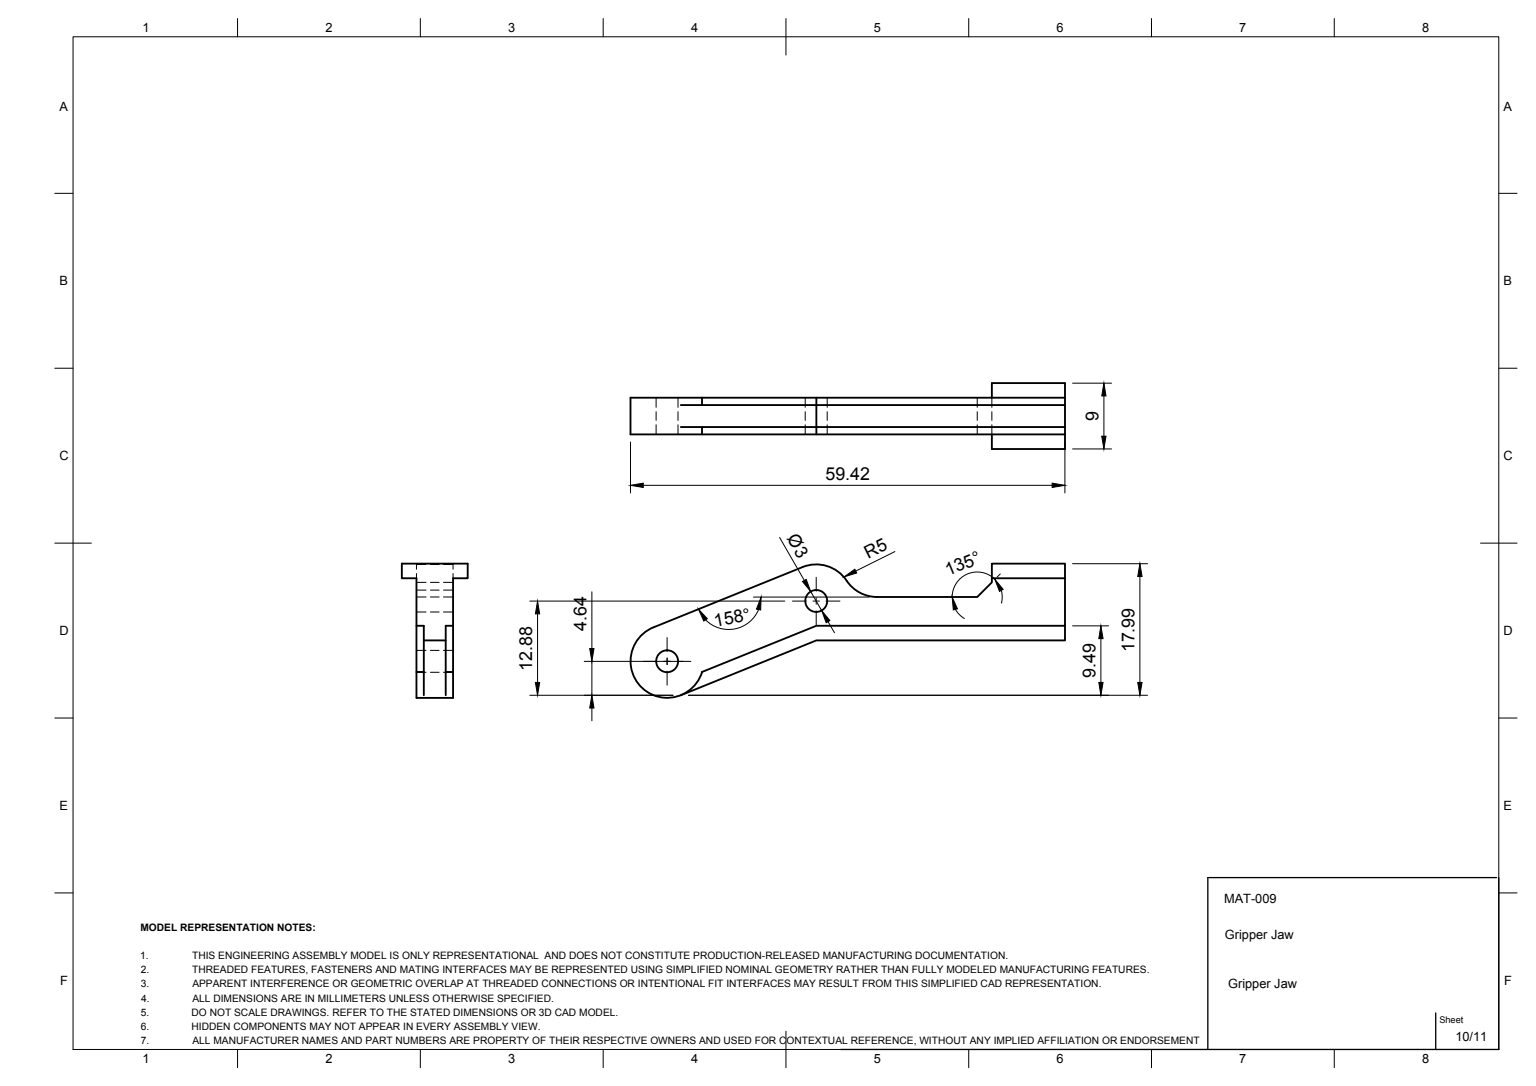
ISO-10303-21;
HEADER;
/* Generated by software containing ST-Developer
 * from STEP Tools, Inc. (www.steptools.com) 
 */

FILE_DESCRIPTION(
/* description */ ('STEP AP214'),
/* implementation_level */ '2;1');

FILE_NAME(
/* name */ 'Gripper Jaw.step',
/* time_stamp */ '2026-11-14T05:43:09-08:00',
/* author */ (''),
/* organization */ (''),
/* preprocessor_version */ 'ST-DEVELOPER v20.2',
/* originating_system */ 'Autodesk Translation Framework v15.17.0.0',
/* authorisation */ '');

FILE_SCHEMA (('AUTOMOTIVE_DESIGN { 1 0 10303 214 3 1 1 }'));
ENDSEC;

DATA;
#10=MECHANICAL_DESIGN_GEOMETRIC_PRESENTATION_REPRESENTATION('',(#150),#11933);
#132=SHAPE_REPRESENTATION_RELATIONSHIP('SRR','None',#11992,#141);
#141=ADVANCED_BREP_SHAPE_REPRESENTATION('',(#159),#11928);
#150=STYLED_ITEM('',(#12043),#159);
#159=MANIFOLD_SOLID_BREP('Body1',#6647);
#194=FACE_BOUND('',#968,.T.);
#195=FACE_BOUND('',#969,.T.);
#196=FACE_BOUND('',#972,.T.);
#197=FACE_BOUND('',#973,.T.);
#256=PLANE('',#7460);
#257=PLANE('',#7463);
#258=PLANE('',#7464);
#259=PLANE('',#7467);
#260=PLANE('',#7468);
#261=PLANE('',#7469);
#262=PLANE('',#7470);
#263=PLANE('',#7471);
#264=PLANE('',#7473);
#265=PLANE('',#7474);
#266=PLANE('',#7475);
#267=PLANE('',#7476);
#268=PLANE('',#7477);
#269=PLANE('',#7478);
#270=PLANE('',#7479);
#271=PLANE('',#7480);
#272=PLANE('',#7481);
#273=PLANE('',#7482);
#274=PLANE('',#7483);
#275=PLANE('',#7484);
#580=FACE_OUTER_BOUND('',#964,.T.);
#581=FACE_OUTER_BOUND('',#965,.T.);
#582=FACE_OUTER_BOUND('',#966,.T.);
#583=FACE_OUTER_BOUND('',#967,.T.);
#584=FACE_OUTER_BOUND('',#970,.T.);
#585=FACE_OUTER_BOUND('',#971,.T.);
#586=FACE_OUTER_BOUND('',#974,.T.);
#587=FACE_OUTER_BOUND('',#975,.T.);
#588=FACE_OUTER_BOUND('',#976,.T.);
#589=FACE_OUTER_BOUND('',#977,.T.);
#590=FACE_OUTER_BOUND('',#978,.T.);
#591=FACE_OUTER_BOUND('',#979,.T.);
#592=FACE_OUTER_BOUND('',#980,.T.);
#593=FACE_OUTER_BOUND('',#981,.T.);
#594=FACE_OUTER_BOUND('',#982,.T.);
#595=FACE_OUTER_BOUND('',#983,.T.);
#596=FACE_OUTER_BOUND('',#984,.T.);
#597=FACE_OUTER_BOUND('',#985,.T.);
#598=FACE_OUTER_BOUND('',#986,.T.);
#599=FACE_OUTER_BOUND('',#987,.T.);
#600=FACE_OUTER_BOUND('',#988,.T.);
#601=FACE_OUTER_BOUND('',#989,.T.);
#602=FACE_OUTER_BOUND('',#990,.T.);
#603=FACE_OUTER_BOUND('',#991,.T.);
#604=FACE_OUTER_BOUND('',#992,.T.);
#964=EDGE_LOOP('',(#5590,#5591,#5592,#5593));
#965=EDGE_LOOP('',(#5594,#5595,#5596,#5597,#5598,#5599,#5600,#5601));
#966=EDGE_LOOP('',(#5602,#5603,#5604,#5605));
#967=EDGE_LOOP('',(#5606,#5607,#5608,#5609,#5610,#5611,#5612,#5613,#5614,
#5615,#5616));
#968=EDGE_LOOP('',(#5617));
#969=EDGE_LOOP('',(#5618));
#970=EDGE_LOOP('',(#5619,#5620,#5621,#5622,#5623,#5624));
#971=EDGE_LOOP('',(#5625,#5626,#5627,#5628,#5629,#5630,#5631,#5632,#5633,
#5634,#5635));
#972=EDGE_LOOP('',(#5636));
#973=EDGE_LOOP('',(#5637));
#974=EDGE_LOOP('',(#5638,#5639,#5640,#5641,#5642,#5643));
#975=EDGE_LOOP('',(#5644,#5645,#5646,#5647));
#976=EDGE_LOOP('',(#5648,#5649,#5650,#5651));
#977=EDGE_LOOP('',(#5652,#5653,#5654,#5655));
#978=EDGE_LOOP('',(#5656,#5657,#5658,#5659));
#979=EDGE_LOOP('',(#5660,#5661,#5662,#5663));
#980=EDGE_LOOP('',(#5664,#5665,#5666,#5667));
#981=EDGE_LOOP('',(#5668,#5669,#5670,#5671));
#982=EDGE_LOOP('',(#5672,#5673,#5674,#5675,#5676,#5677,#5678,#5679));
#983=EDGE_LOOP('',(#5680,#5681,#5682,#5683));
#984=EDGE_LOOP('',(#5684,#5685,#5686,#5687,#5688,#5689,#5690,#5691,#5692,
#5693,#5694,#5695));
#985=EDGE_LOOP('',(#5696,#5697,#5698,#5699));
#986=EDGE_LOOP('',(#5700,#5701,#5702,#5703));
#987=EDGE_LOOP('',(#5704,#5705,#5706,#5707));
#988=EDGE_LOOP('',(#5708,#5709,#5710,#5711));
#989=EDGE_LOOP('',(#5712,#5713,#5714,#5715));
#990=EDGE_LOOP('',(#5716,#5717,#5718,#5719));
#991=EDGE_LOOP('',(#5720,#5721,#5722,#5723));
#992=EDGE_LOOP('',(#5724,#5725,#5726,#5727));
#1381=LINE('',#11410,#1843);
#1382=LINE('',#11417,#1844);
#1383=LINE('',#11421,#1845);
#1384=LINE('',#11425,#1846);
#1385=LINE('',#11428,#1847);
#1386=LINE('',#11433,#1848);
#1387=LINE('',#11438,#1849);
#1388=LINE('',#11440,#1850);
#1389=LINE('',#11442,#1851);
#1390=LINE('',#11444,#1852);
#1391=LINE('',#11445,#1853);
#1392=LINE('',#11447,#1854);
#1393=LINE('',#11453,#1855);
#1394=LINE('',#11454,#1856);
#1395=LINE('',#11457,#1857);
#1396=LINE('',#11459,#1858);
#1397=LINE('',#11461,#1859);
#1398=LINE('',#11463,#1860);
#1399=LINE('',#11464,#1861);
#1400=LINE('',#11468,#1862);
#1401=LINE('',#11470,#1863);
#1402=LINE('',#11472,#1864);
#1403=LINE('',#11474,#1865);
#1404=LINE('',#11479,#1866);
#1405=LINE('',#11481,#1867);
#1406=LINE('',#11483,#1868);
#1407=LINE('',#11484,#1869);
#1408=LINE('',#11488,#1870);
#1409=LINE('',#11489,#1871);
#1410=LINE('',#11491,#1872);
#1411=LINE('',#11493,#1873);
#1412=LINE('',#11494,#1874);
#1413=LINE('',#11496,#1875);
#1414=LINE('',#11498,#1876);
#1415=LINE('',#11500,#1877);
#1416=LINE('',#11502,#1878);
#1417=LINE('',#11504,#1879);
#1418=LINE('',#11506,#1880);
#1419=LINE('',#11507,#1881);
#1420=LINE('',#11509,#1882);
#1421=LINE('',#11512,#1883);
#1422=LINE('',#11514,#1884);
#1423=LINE('',#11516,#1885);
#1424=LINE('',#11518,#1886);
#1425=LINE('',#11519,#1887);
#1426=LINE('',#11522,#1888);
#1427=LINE('',#11524,#1889);
#1428=LINE('',#11525,#1890);
#1429=LINE('',#11527,#1891);
#1430=LINE('',#11529,#1892);
#1431=LINE('',#11530,#1893);
#1432=LINE('',#11532,#1894);
#1433=LINE('',#11533,#1895);
#1434=LINE('',#11534,#1896);
#1435=LINE('',#11535,#1897);
#1436=LINE('',#11540,#1898);
#1437=LINE('',#11543,#1899);
#1843=VECTOR('',#9357,1.5);
#1844=VECTOR('',#9364,1000.);
#1845=VECTOR('',#9367,1000.);
#1846=VECTOR('',#9370,1000.);
#1847=VECTOR('',#9373,1000.);
#1848=VECTOR('',#9378,1.5);
#1849=VECTOR('',#9383,1000.);
#1850=VECTOR('',#9384,1000.);
#1851=VECTOR('',#9385,1000.);
#1852=VECTOR('',#9386,1000.);
#1853=VECTOR('',#9387,1000.);
#1854=VECTOR('',#9388,1000.);
#1855=VECTOR('',#9393,1000.);
#1856=VECTOR('',#9394,1000.);
#1857=VECTOR('',#9397,1000.);
#1858=VECTOR('',#9398,1000.);
#1859=VECTOR('',#9399,1000.);
#1860=VECTOR('',#9400,1000.);
#1861=VECTOR('',#9401,1000.);
#1862=VECTOR('',#9404,1000.);
#1863=VECTOR('',#9405,1000.);
#1864=VECTOR('',#9406,1000.);
#1865=VECTOR('',#9407,1000.);
#1866=VECTOR('',#9412,1000.);
#1867=VECTOR('',#9413,1000.);
#1868=VECTOR('',#9414,1000.);
#1869=VECTOR('',#9415,1000.);
#1870=VECTOR('',#9418,1000.);
#1871=VECTOR('',#9419,1000.);
#1872=VECTOR('',#9420,1000.);
#1873=VECTOR('',#9421,1000.);
#1874=VECTOR('',#9422,1000.);
#1875=VECTOR('',#9425,1000.);
#1876=VECTOR('',#9428,1000.);
#1877=VECTOR('',#9431,1000.);
#1878=VECTOR('',#9434,1000.);
#1879=VECTOR('',#9437,1000.);
#1880=VECTOR('',#9440,1000.);
#1881=VECTOR('',#9441,1000.);
#1882=VECTOR('',#9444,1000.);
#1883=VECTOR('',#9447,1000.);
#1884=VECTOR('',#9448,1000.);
#1885=VECTOR('',#9449,1000.);
#1886=VECTOR('',#9450,1000.);
#1887=VECTOR('',#9451,1000.);
#1888=VECTOR('',#9454,1000.);
#1889=VECTOR('',#9455,1000.);
#1890=VECTOR('',#9456,1000.);
#1891=VECTOR('',#9459,1000.);
#1892=VECTOR('',#9460,1000.);
#1893=VECTOR('',#9461,1000.);
#1894=VECTOR('',#9462,1000.);
#1895=VECTOR('',#9463,1000.);
#1896=VECTOR('',#9464,1000.);
#1897=VECTOR('',#9465,1000.);
#1898=VECTOR('',#9474,1000.);
#1899=VECTOR('',#9479,1000.);
#2426=CIRCLE('',#7450,1.5);
#2427=CIRCLE('',#7451,1.5);
#2428=CIRCLE('',#7453,5.);
#2429=CIRCLE('',#7454,5.);
#2430=CIRCLE('',#7455,5.);
#2431=CIRCLE('',#7456,5.);
#2432=CIRCLE('',#7458,1.5);
#2433=CIRCLE('',#7459,1.5);
#2434=CIRCLE('',#7461,5.);
#2435=CIRCLE('',#7462,5.);
#2436=CIRCLE('',#7465,5.);
#2437=CIRCLE('',#7466,5.);
#2993=VERTEX_POINT('',#11407);
#2994=VERTEX_POINT('',#11409);
#2995=VERTEX_POINT('',#11413);
#2996=VERTEX_POINT('',#11414);
#2997=VERTEX_POINT('',#11416);
#2998=VERTEX_POINT('',#11418);
#2999=VERTEX_POINT('',#11420);
#3000=VERTEX_POINT('',#11422);
#3001=VERTEX_POINT('',#11424);
#3002=VERTEX_POINT('',#11426);
#3003=VERTEX_POINT('',#11430);
#3004=VERTEX_POINT('',#11432);
#3005=VERTEX_POINT('',#11436);
#3006=VERTEX_POINT('',#11437);
#3007=VERTEX_POINT('',#11439);
#3008=VERTEX_POINT('',#11441);
#3009=VERTEX_POINT('',#11443);
#3010=VERTEX_POINT('',#11446);
#3011=VERTEX_POINT('',#11448);
#3012=VERTEX_POINT('',#11450);
#3013=VERTEX_POINT('',#11452);
#3014=VERTEX_POINT('',#11456);
#3015=VERTEX_POINT('',#11458);
#3016=VERTEX_POINT('',#11460);
#3017=VERTEX_POINT('',#11462);
#3018=VERTEX_POINT('',#11466);
#3019=VERTEX_POINT('',#11467);
#3020=VERTEX_POINT('',#11469);
#3021=VERTEX_POINT('',#11471);
#3022=VERTEX_POINT('',#11473);
#3023=VERTEX_POINT('',#11475);
#3024=VERTEX_POINT('',#11477);
#3025=VERTEX_POINT('',#11480);
#3026=VERTEX_POINT('',#11482);
#3027=VERTEX_POINT('',#11486);
#3028=VERTEX_POINT('',#11487);
#3029=VERTEX_POINT('',#11490);
#3030=VERTEX_POINT('',#11492);
#3031=VERTEX_POINT('',#11511);
#3032=VERTEX_POINT('',#11513);
#3033=VERTEX_POINT('',#11515);
#3034=VERTEX_POINT('',#11517);
#3035=VERTEX_POINT('',#11521);
#3036=VERTEX_POINT('',#11523);
#3037=VERTEX_POINT('',#11528);
#3038=VERTEX_POINT('',#11531);
#3884=EDGE_CURVE('',#2993,#2993,#2426,.T.);
#3885=EDGE_CURVE('',#2993,#2994,#1381,.T.);
#3886=EDGE_CURVE('',#2994,#2994,#2427,.T.);
#3887=EDGE_CURVE('',#2995,#2996,#2428,.T.);
#3888=EDGE_CURVE('',#2995,#2997,#1382,.T.);
#3889=EDGE_CURVE('',#2997,#2998,#2429,.T.);
#3890=EDGE_CURVE('',#2998,#2999,#1383,.T.);
#3891=EDGE_CURVE('',#3000,#2999,#2430,.T.);
#3892=EDGE_CURVE('',#3001,#3000,#1384,.T.);
#3893=EDGE_CURVE('',#3001,#3002,#2431,.T.);
#3894=EDGE_CURVE('',#2996,#3002,#1385,.T.);
#3895=EDGE_CURVE('',#3003,#3003,#2432,.T.);
#3896=EDGE_CURVE('',#3003,#3004,#1386,.T.);
#3897=EDGE_CURVE('',#3004,#3004,#2433,.T.);
#3898=EDGE_CURVE('',#3005,#3006,#1387,.T.);
#3899=EDGE_CURVE('',#3006,#3007,#1388,.T.);
#3900=EDGE_CURVE('',#3007,#3008,#1389,.T.);
#3901=EDGE_CURVE('',#3008,#3009,#1390,.T.);
#3902=EDGE_CURVE('',#3009,#2995,#1391,.T.);
#3903=EDGE_CURVE('',#2996,#3010,#1392,.T.);
#3904=EDGE_CURVE('',#3010,#3011,#2434,.T.);
#3905=EDGE_CURVE('',#3011,#3012,#2435,.T.);
#3906=EDGE_CURVE('',#3012,#3013,#1393,.T.);
#3907=EDGE_CURVE('',#3013,#3005,#1394,.T.);
#3908=EDGE_CURVE('',#3014,#2997,#1395,.T.);
#3909=EDGE_CURVE('',#3014,#3015,#1396,.T.);
#3910=EDGE_CURVE('',#3016,#3015,#1397,.T.);
#3911=EDGE_CURVE('',#3017,#3016,#1398,.T.);
#3912=EDGE_CURVE('',#3017,#2998,#1399,.T.);
#3913=EDGE_CURVE('',#3018,#3019,#1400,.T.);
#3914=EDGE_CURVE('',#3020,#3018,#1401,.T.);
#3915=EDGE_CURVE('',#3021,#3020,#1402,.T.);
#3916=EDGE_CURVE('',#3022,#3021,#1403,.T.);
#3917=EDGE_CURVE('',#3022,#3023,#2436,.T.);
#3918=EDGE_CURVE('',#3024,#3023,#2437,.T.);
#3919=EDGE_CURVE('',#3002,#3024,#1404,.T.);
#3920=EDGE_CURVE('',#3025,#3001,#1405,.T.);
#3921=EDGE_CURVE('',#3026,#3025,#1406,.T.);
#3922=EDGE_CURVE('',#3019,#3026,#1407,.T.);
#3923=EDGE_CURVE('',#3027,#3028,#1408,.T.);
#3924=EDGE_CURVE('',#3028,#3000,#1409,.T.);
#3925=EDGE_CURVE('',#3029,#2999,#1410,.T.);
#3926=EDGE_CURVE('',#3029,#3030,#1411,.T.);
#3927=EDGE_CURVE('',#3030,#3027,#1412,.T.);
#3928=EDGE_CURVE('',#3009,#3014,#1413,.T.);
#3929=EDGE_CURVE('',#3025,#3028,#1414,.T.);
#3930=EDGE_CURVE('',#3010,#3024,#1415,.T.);
#3931=EDGE_CURVE('',#3017,#3029,#1416,.T.);
#3932=EDGE_CURVE('',#3023,#3011,#1417,.T.);
#3933=EDGE_CURVE('',#3012,#3022,#1418,.T.);
#3934=EDGE_CURVE('',#3013,#3021,#1419,.T.);
#3935=EDGE_CURVE('',#3005,#3020,#1420,.T.);
#3936=EDGE_CURVE('',#3031,#3018,#1421,.T.);
#3937=EDGE_CURVE('',#3031,#3032,#1422,.T.);
#3938=EDGE_CURVE('',#3033,#3032,#1423,.T.);
#3939=EDGE_CURVE('',#3034,#3033,#1424,.T.);
#3940=EDGE_CURVE('',#3034,#3006,#1425,.T.);
#3941=EDGE_CURVE('',#3032,#3035,#1426,.T.);
#3942=EDGE_CURVE('',#3036,#3035,#1427,.T.);
#3943=EDGE_CURVE('',#3033,#3036,#1428,.T.);
#3944=EDGE_CURVE('',#3008,#3015,#1429,.T.);
#3945=EDGE_CURVE('',#3037,#3007,#1430,.T.);
#3946=EDGE_CURVE('',#3036,#3037,#1431,.T.);
#3947=EDGE_CURVE('',#3035,#3038,#1432,.T.);
#3948=EDGE_CURVE('',#3038,#3019,#1433,.T.);
#3949=EDGE_CURVE('',#3026,#3027,#1434,.T.);
#3950=EDGE_CURVE('',#3016,#3030,#1435,.T.);
#3951=EDGE_CURVE('',#3034,#3037,#1436,.T.);
#3952=EDGE_CURVE('',#3031,#3038,#1437,.T.);
#5590=ORIENTED_EDGE('',*,*,#3884,.T.);
#5591=ORIENTED_EDGE('',*,*,#3885,.T.);
#5592=ORIENTED_EDGE('',*,*,#3886,.F.);
#5593=ORIENTED_EDGE('',*,*,#3885,.F.);
#5594=ORIENTED_EDGE('',*,*,#3887,.F.);
#5595=ORIENTED_EDGE('',*,*,#3888,.T.);
#5596=ORIENTED_EDGE('',*,*,#3889,.T.);
#5597=ORIENTED_EDGE('',*,*,#3890,.T.);
#5598=ORIENTED_EDGE('',*,*,#3891,.F.);
#5599=ORIENTED_EDGE('',*,*,#3892,.F.);
#5600=ORIENTED_EDGE('',*,*,#3893,.T.);
#5601=ORIENTED_EDGE('',*,*,#3894,.F.);
#5602=ORIENTED_EDGE('',*,*,#3895,.T.);
#5603=ORIENTED_EDGE('',*,*,#3896,.T.);
#5604=ORIENTED_EDGE('',*,*,#3897,.F.);
#5605=ORIENTED_EDGE('',*,*,#3896,.F.);
#5606=ORIENTED_EDGE('',*,*,#3898,.T.);
#5607=ORIENTED_EDGE('',*,*,#3899,.T.);
#5608=ORIENTED_EDGE('',*,*,#3900,.T.);
#5609=ORIENTED_EDGE('',*,*,#3901,.T.);
#5610=ORIENTED_EDGE('',*,*,#3902,.T.);
#5611=ORIENTED_EDGE('',*,*,#3887,.T.);
#5612=ORIENTED_EDGE('',*,*,#3903,.T.);
#5613=ORIENTED_EDGE('',*,*,#3904,.T.);
#5614=ORIENTED_EDGE('',*,*,#3905,.T.);
#5615=ORIENTED_EDGE('',*,*,#3906,.T.);
#5616=ORIENTED_EDGE('',*,*,#3907,.T.);
#5617=ORIENTED_EDGE('',*,*,#3884,.F.);
#5618=ORIENTED_EDGE('',*,*,#3895,.F.);
#5619=ORIENTED_EDGE('',*,*,#3908,.F.);
#5620=ORIENTED_EDGE('',*,*,#3909,.T.);
#5621=ORIENTED_EDGE('',*,*,#3910,.F.);
#5622=ORIENTED_EDGE('',*,*,#3911,.F.);
#5623=ORIENTED_EDGE('',*,*,#3912,.T.);
#5624=ORIENTED_EDGE('',*,*,#3889,.F.);
#5625=ORIENTED_EDGE('',*,*,#3913,.F.);
#5626=ORIENTED_EDGE('',*,*,#3914,.F.);
#5627=ORIENTED_EDGE('',*,*,#3915,.F.);
#5628=ORIENTED_EDGE('',*,*,#3916,.F.);
#5629=ORIENTED_EDGE('',*,*,#3917,.T.);
#5630=ORIENTED_EDGE('',*,*,#3918,.F.);
#5631=ORIENTED_EDGE('',*,*,#3919,.F.);
#5632=ORIENTED_EDGE('',*,*,#3893,.F.);
#5633=ORIENTED_EDGE('',*,*,#3920,.F.);
#5634=ORIENTED_EDGE('',*,*,#3921,.F.);
#5635=ORIENTED_EDGE('',*,*,#3922,.F.);
#5636=ORIENTED_EDGE('',*,*,#3897,.T.);
#5637=ORIENTED_EDGE('',*,*,#3886,.T.);
#5638=ORIENTED_EDGE('',*,*,#3923,.T.);
#5639=ORIENTED_EDGE('',*,*,#3924,.T.);
#5640=ORIENTED_EDGE('',*,*,#3891,.T.);
#5641=ORIENTED_EDGE('',*,*,#3925,.F.);
#5642=ORIENTED_EDGE('',*,*,#3926,.T.);
#5643=ORIENTED_EDGE('',*,*,#3927,.T.);
#5644=ORIENTED_EDGE('',*,*,#3902,.F.);
#5645=ORIENTED_EDGE('',*,*,#3928,.T.);
#5646=ORIENTED_EDGE('',*,*,#3908,.T.);
#5647=ORIENTED_EDGE('',*,*,#3888,.F.);
#5648=ORIENTED_EDGE('',*,*,#3924,.F.);
#5649=ORIENTED_EDGE('',*,*,#3929,.F.);
#5650=ORIENTED_EDGE('',*,*,#3920,.T.);
#5651=ORIENTED_EDGE('',*,*,#3892,.T.);
#5652=ORIENTED_EDGE('',*,*,#3919,.T.);
#5653=ORIENTED_EDGE('',*,*,#3930,.F.);
#5654=ORIENTED_EDGE('',*,*,#3903,.F.);
#5655=ORIENTED_EDGE('',*,*,#3894,.T.);
#5656=ORIENTED_EDGE('',*,*,#3931,.T.);
#5657=ORIENTED_EDGE('',*,*,#3925,.T.);
#5658=ORIENTED_EDGE('',*,*,#3890,.F.);
#5659=ORIENTED_EDGE('',*,*,#3912,.F.);
#5660=ORIENTED_EDGE('',*,*,#3918,.T.);
#5661=ORIENTED_EDGE('',*,*,#3932,.T.);
#5662=ORIENTED_EDGE('',*,*,#3904,.F.);
#5663=ORIENTED_EDGE('',*,*,#3930,.T.);
#5664=ORIENTED_EDGE('',*,*,#3906,.F.);
#5665=ORIENTED_EDGE('',*,*,#3933,.T.);
#5666=ORIENTED_EDGE('',*,*,#3916,.T.);
#5667=ORIENTED_EDGE('',*,*,#3934,.F.);
#5668=ORIENTED_EDGE('',*,*,#3915,.T.);
#5669=ORIENTED_EDGE('',*,*,#3935,.F.);
#5670=ORIENTED_EDGE('',*,*,#3907,.F.);
#5671=ORIENTED_EDGE('',*,*,#3934,.T.);
#5672=ORIENTED_EDGE('',*,*,#3914,.T.);
#5673=ORIENTED_EDGE('',*,*,#3936,.F.);
#5674=ORIENTED_EDGE('',*,*,#3937,.T.);
#5675=ORIENTED_EDGE('',*,*,#3938,.F.);
#5676=ORIENTED_EDGE('',*,*,#3939,.F.);
#5677=ORIENTED_EDGE('',*,*,#3940,.T.);
#5678=ORIENTED_EDGE('',*,*,#3898,.F.);
#5679=ORIENTED_EDGE('',*,*,#3935,.T.);
#5680=ORIENTED_EDGE('',*,*,#3938,.T.);
#5681=ORIENTED_EDGE('',*,*,#3941,.T.);
#5682=ORIENTED_EDGE('',*,*,#3942,.F.);
#5683=ORIENTED_EDGE('',*,*,#3943,.F.);
#5684=ORIENTED_EDGE('',*,*,#3910,.T.);
#5685=ORIENTED_EDGE('',*,*,#3944,.F.);
#5686=ORIENTED_EDGE('',*,*,#3900,.F.);
#5687=ORIENTED_EDGE('',*,*,#3945,.F.);
#5688=ORIENTED_EDGE('',*,*,#3946,.F.);
#5689=ORIENTED_EDGE('',*,*,#3942,.T.);
#5690=ORIENTED_EDGE('',*,*,#3947,.T.);
#5691=ORIENTED_EDGE('',*,*,#3948,.T.);
#5692=ORIENTED_EDGE('',*,*,#3922,.T.);
#5693=ORIENTED_EDGE('',*,*,#3949,.T.);
#5694=ORIENTED_EDGE('',*,*,#3927,.F.);
#5695=ORIENTED_EDGE('',*,*,#3950,.F.);
#5696=ORIENTED_EDGE('',*,*,#3926,.F.);
#5697=ORIENTED_EDGE('',*,*,#3931,.F.);
#5698=ORIENTED_EDGE('',*,*,#3911,.T.);
#5699=ORIENTED_EDGE('',*,*,#3950,.T.);
#5700=ORIENTED_EDGE('',*,*,#3909,.F.);
#5701=ORIENTED_EDGE('',*,*,#3928,.F.);
#5702=ORIENTED_EDGE('',*,*,#3901,.F.);
#5703=ORIENTED_EDGE('',*,*,#3944,.T.);
#5704=ORIENTED_EDGE('',*,*,#3923,.F.);
#5705=ORIENTED_EDGE('',*,*,#3949,.F.);
#5706=ORIENTED_EDGE('',*,*,#3921,.T.);
#5707=ORIENTED_EDGE('',*,*,#3929,.T.);
#5708=ORIENTED_EDGE('',*,*,#3899,.F.);
#5709=ORIENTED_EDGE('',*,*,#3940,.F.);
#5710=ORIENTED_EDGE('',*,*,#3951,.T.);
#5711=ORIENTED_EDGE('',*,*,#3945,.T.);
#5712=ORIENTED_EDGE('',*,*,#3951,.F.);
#5713=ORIENTED_EDGE('',*,*,#3939,.T.);
#5714=ORIENTED_EDGE('',*,*,#3943,.T.);
#5715=ORIENTED_EDGE('',*,*,#3946,.T.);
#5716=ORIENTED_EDGE('',*,*,#3913,.T.);
#5717=ORIENTED_EDGE('',*,*,#3948,.F.);
#5718=ORIENTED_EDGE('',*,*,#3952,.F.);
#5719=ORIENTED_EDGE('',*,*,#3936,.T.);
#5720=ORIENTED_EDGE('',*,*,#3952,.T.);
#5721=ORIENTED_EDGE('',*,*,#3947,.F.);
#5722=ORIENTED_EDGE('',*,*,#3941,.F.);
#5723=ORIENTED_EDGE('',*,*,#3937,.F.);
#5724=ORIENTED_EDGE('',*,*,#3905,.F.);
#5725=ORIENTED_EDGE('',*,*,#3932,.F.);
#5726=ORIENTED_EDGE('',*,*,#3917,.F.);
#5727=ORIENTED_EDGE('',*,*,#3933,.F.);
#6260=CYLINDRICAL_SURFACE('',#7449,1.5);
#6261=CYLINDRICAL_SURFACE('',#7452,5.);
#6262=CYLINDRICAL_SURFACE('',#7457,1.5);
#6263=CYLINDRICAL_SURFACE('',#7472,5.);
#6264=CYLINDRICAL_SURFACE('',#7485,5.);
#6550=ADVANCED_FACE('',(#580),#6260,.F.);
#6551=ADVANCED_FACE('',(#581),#6261,.T.);
#6552=ADVANCED_FACE('',(#582),#6262,.F.);
#6553=ADVANCED_FACE('',(#583,#194,#195),#256,.T.);
#6554=ADVANCED_FACE('',(#584),#257,.T.);
#6555=ADVANCED_FACE('',(#585,#196,#197),#258,.T.);
#6556=ADVANCED_FACE('',(#586),#259,.F.);
#6557=ADVANCED_FACE('',(#587),#260,.F.);
#6558=ADVANCED_FACE('',(#588),#261,.T.);
#6559=ADVANCED_FACE('',(#589),#262,.F.);
#6560=ADVANCED_FACE('',(#590),#263,.F.);
#6561=ADVANCED_FACE('',(#591),#6263,.T.);
#6562=ADVANCED_FACE('',(#592),#264,.T.);
#6563=ADVANCED_FACE('',(#593),#265,.F.);
#6564=ADVANCED_FACE('',(#594),#266,.T.);
#6565=ADVANCED_FACE('',(#595),#267,.T.);
#6566=ADVANCED_FACE('',(#596),#268,.T.);
#6567=ADVANCED_FACE('',(#597),#269,.T.);
#6568=ADVANCED_FACE('',(#598),#270,.F.);
#6569=ADVANCED_FACE('',(#599),#271,.T.);
#6570=ADVANCED_FACE('',(#600),#272,.T.);
#6571=ADVANCED_FACE('',(#601),#273,.T.);
#6572=ADVANCED_FACE('',(#602),#274,.F.);
#6573=ADVANCED_FACE('',(#603),#275,.T.);
#6574=ADVANCED_FACE('',(#604),#6264,.F.);
#6647=CLOSED_SHELL('',(#6550,#6551,#6552,#6553,#6554,#6555,#6556,#6557,
#6558,#6559,#6560,#6561,#6562,#6563,#6564,#6565,#6566,#6567,#6568,#6569,
#6570,#6571,#6572,#6573,#6574));
#7448=AXIS2_PLACEMENT_3D('',#11405,#9351,#9352);
#7449=AXIS2_PLACEMENT_3D('',#11406,#9353,#9354);
#7450=AXIS2_PLACEMENT_3D('',#11408,#9355,#9356);
#7451=AXIS2_PLACEMENT_3D('',#11411,#9358,#9359);
#7452=AXIS2_PLACEMENT_3D('',#11412,#9360,#9361);
#7453=AXIS2_PLACEMENT_3D('',#11415,#9362,#9363);
#7454=AXIS2_PLACEMENT_3D('',#11419,#9365,#9366);
#7455=AXIS2_PLACEMENT_3D('',#11423,#9368,#9369);
#7456=AXIS2_PLACEMENT_3D('',#11427,#9371,#9372);
#7457=AXIS2_PLACEMENT_3D('',#11429,#9374,#9375);
#7458=AXIS2_PLACEMENT_3D('',#11431,#9376,#9377);
#7459=AXIS2_PLACEMENT_3D('',#11434,#9379,#9380);
#7460=AXIS2_PLACEMENT_3D('',#11435,#9381,#9382);
#7461=AXIS2_PLACEMENT_3D('',#11449,#9389,#9390);
#7462=AXIS2_PLACEMENT_3D('',#11451,#9391,#9392);
#7463=AXIS2_PLACEMENT_3D('',#11455,#9395,#9396);
#7464=AXIS2_PLACEMENT_3D('',#11465,#9402,#9403);
#7465=AXIS2_PLACEMENT_3D('',#11476,#9408,#9409);
#7466=AXIS2_PLACEMENT_3D('',#11478,#9410,#9411);
#7467=AXIS2_PLACEMENT_3D('',#11485,#9416,#9417);
#7468=AXIS2_PLACEMENT_3D('',#11495,#9423,#9424);
#7469=AXIS2_PLACEMENT_3D('',#11497,#9426,#9427);
#7470=AXIS2_PLACEMENT_3D('',#11499,#9429,#9430);
#7471=AXIS2_PLACEMENT_3D('',#11501,#9432,#9433);
#7472=AXIS2_PLACEMENT_3D('',#11503,#9435,#9436);
#7473=AXIS2_PLACEMENT_3D('',#11505,#9438,#9439);
#7474=AXIS2_PLACEMENT_3D('',#11508,#9442,#9443);
#7475=AXIS2_PLACEMENT_3D('',#11510,#9445,#9446);
#7476=AXIS2_PLACEMENT_3D('',#11520,#9452,#9453);
#7477=AXIS2_PLACEMENT_3D('',#11526,#9457,#9458);
#7478=AXIS2_PLACEMENT_3D('',#11536,#9466,#9467);
#7479=AXIS2_PLACEMENT_3D('',#11537,#9468,#9469);
#7480=AXIS2_PLACEMENT_3D('',#11538,#9470,#9471);
#7481=AXIS2_PLACEMENT_3D('',#11539,#9472,#9473);
#7482=AXIS2_PLACEMENT_3D('',#11541,#9475,#9476);
#7483=AXIS2_PLACEMENT_3D('',#11542,#9477,#9478);
#7484=AXIS2_PLACEMENT_3D('',#11544,#9480,#9481);
#7485=AXIS2_PLACEMENT_3D('',#11545,#9482,#9483);
#9351=DIRECTION('axis',(0.,0.,1.));
#9352=DIRECTION('refdir',(1.,0.,0.));
#9353=DIRECTION('center_axis',(0.,0.,-1.));
#9354=DIRECTION('ref_axis',(-1.,0.,0.));
#9355=DIRECTION('center_axis',(0.,0.,1.));
#9356=DIRECTION('ref_axis',(1.,0.,0.));
#9357=DIRECTION('',(0.,0.,-1.));
#9358=DIRECTION('center_axis',(0.,0.,1.));
#9359=DIRECTION('ref_axis',(1.,0.,0.));
#9360=DIRECTION('center_axis',(0.,0.,-1.));
#9361=DIRECTION('ref_axis',(-1.,0.,0.));
#9362=DIRECTION('center_axis',(0.,0.,1.));
#9363=DIRECTION('ref_axis',(1.,0.,0.));
#9364=DIRECTION('',(0.,0.,-1.));
#9365=DIRECTION('center_axis',(0.,0.,1.));
#9366=DIRECTION('ref_axis',(1.,0.,0.));
#9367=DIRECTION('',(0.,0.,-1.));
#9368=DIRECTION('center_axis',(0.,0.,1.));
#9369=DIRECTION('ref_axis',(1.,0.,0.));
#9370=DIRECTION('',(0.,0.,1.));
#9371=DIRECTION('center_axis',(0.,0.,1.));
#9372=DIRECTION('ref_axis',(1.,0.,0.));
#9373=DIRECTION('',(0.,0.,-1.));
#9374=DIRECTION('center_axis',(0.,0.,-1.));
#9375=DIRECTION('ref_axis',(-1.,0.,0.));
#9376=DIRECTION('center_axis',(0.,0.,1.));
#9377=DIRECTION('ref_axis',(1.,0.,0.));
#9378=DIRECTION('',(0.,0.,-1.));
#9379=DIRECTION('center_axis',(0.,0.,1.));
#9380=DIRECTION('ref_axis',(1.,0.,0.));
#9381=DIRECTION('center_axis',(0.,0.,1.));
#9382=DIRECTION('ref_axis',(1.,0.,0.));
#9383=DIRECTION('',(0.374606593415916,-0.927183854566786,0.));
#9384=DIRECTION('',(0.927183854566785,0.374606593415917,0.));
#9385=DIRECTION('',(-0.374606593415917,0.927183854566785,0.));
#9386=DIRECTION('',(-0.927183854566787,-0.374606593415913,0.));
#9387=DIRECTION('',(-1.,0.,0.));
#9388=DIRECTION('',(1.,0.,0.));
#9389=DIRECTION('center_axis',(0.,0.,1.));
#9390=DIRECTION('ref_axis',(1.,0.,0.));
#9391=DIRECTION('center_axis',(0.,0.,-1.));
#9392=DIRECTION('ref_axis',(1.,0.,0.));
#9393=DIRECTION('',(0.927183854566786,0.374606593415915,0.));
#9394=DIRECTION('',(0.920504853452439,-0.390731128489277,0.));
#9395=DIRECTION('center_axis',(0.,0.,1.));
#9396=DIRECTION('ref_axis',(1.,0.,0.));
#9397=DIRECTION('',(-1.,0.,0.));
#9398=DIRECTION('',(0.927183854566787,0.374606593415913,0.));
#9399=DIRECTION('',(0.374606593415916,-0.927183854566786,0.));
#9400=DIRECTION('',(0.927183854566787,0.374606593415913,0.));
#9401=DIRECTION('',(-1.,0.,0.));
#9402=DIRECTION('center_axis',(0.,0.,-1.));
#9403=DIRECTION('ref_axis',(1.,0.,0.));
#9404=DIRECTION('',(0.927183854566785,0.374606593415917,0.));
#9405=DIRECTION('',(0.374606593415916,-0.927183854566786,0.));
#9406=DIRECTION('',(0.920504853452439,-0.390731128489277,0.));
#9407=DIRECTION('',(0.927183854566786,0.374606593415915,0.));
#9408=DIRECTION('center_axis',(0.,0.,1.));
#9409=DIRECTION('ref_axis',(-1.,-5.29090660172926E-15,0.));
#9410=DIRECTION('center_axis',(0.,0.,1.));
#9411=DIRECTION('ref_axis',(1.,0.,0.));
#9412=DIRECTION('',(1.,0.,0.));
#9413=DIRECTION('',(-1.,0.,0.));
#9414=DIRECTION('',(-0.927183854566787,-0.374606593415913,0.));
#9415=DIRECTION('',(-0.374606593415917,0.927183854566785,0.));
#9416=DIRECTION('center_axis',(0.,0.,1.));
#9417=DIRECTION('ref_axis',(1.,0.,0.));
#9418=DIRECTION('',(-0.927183854566787,-0.374606593415913,0.));
#9419=DIRECTION('',(-1.,0.,0.));
#9420=DIRECTION('',(-1.,0.,0.));
#9421=DIRECTION('',(0.927183854566787,0.374606593415913,0.));
#9422=DIRECTION('',(0.374606593415916,-0.927183854566786,0.));
#9423=DIRECTION('center_axis',(0.,-1.,0.));
#9424=DIRECTION('ref_axis',(0.,0.,-1.));
#9425=DIRECTION('',(0.,0.,-1.));
#9426=DIRECTION('center_axis',(0.,1.,0.));
#9427=DIRECTION('ref_axis',(0.,0.,1.));
#9428=DIRECTION('',(0.,0.,1.));
#9429=DIRECTION('center_axis',(0.,1.,0.));
#9430=DIRECTION('ref_axis',(0.,0.,1.));
#9431=DIRECTION('',(0.,0.,-1.));
#9432=DIRECTION('center_axis',(0.,-1.,0.));
#9433=DIRECTION('ref_axis',(0.,0.,-1.));
#9434=DIRECTION('',(0.,0.,-1.));
#9435=DIRECTION('center_axis',(0.,0.,-1.));
#9436=DIRECTION('ref_axis',(-1.,0.,0.));
#9437=DIRECTION('',(0.,0.,1.));
#9438=DIRECTION('center_axis',(0.374606593415915,-0.927183854566786,0.));
#9439=DIRECTION('ref_axis',(0.927183854566786,0.374606593415915,0.));
#9440=DIRECTION('',(0.,0.,-1.));
#9441=DIRECTION('',(0.,0.,-1.));
#9442=DIRECTION('center_axis',(0.390731128489276,0.920504853452439,0.));
#9443=DIRECTION('ref_axis',(-0.920504853452439,0.390731128489276,0.));
#9444=DIRECTION('',(0.,0.,-1.));
#9445=DIRECTION('center_axis',(-0.927183854566787,-0.374606593415913,0.));
#9446=DIRECTION('ref_axis',(0.374606593415913,-0.927183854566787,0.));
#9447=DIRECTION('',(0.,0.,1.));
#9448=DIRECTION('',(0.374606593415916,-0.927183854566786,0.));
#9449=DIRECTION('',(0.,0.,-1.));
#9450=DIRECTION('',(0.374606593415916,-0.927183854566786,0.));
#9451=DIRECTION('',(0.,0.,-1.));
#9452=DIRECTION('center_axis',(0.374606593415915,-0.927183854566786,0.));
#9453=DIRECTION('ref_axis',(0.927183854566786,0.374606593415915,0.));
#9454=DIRECTION('',(0.927183854566786,0.374606593415915,0.));
#9455=DIRECTION('',(0.,0.,-1.));
#9456=DIRECTION('',(0.927183854566786,0.374606593415915,0.));
#9457=DIRECTION('center_axis',(0.927183854566786,0.374606593415916,0.));
#9458=DIRECTION('ref_axis',(-0.374606593415916,0.927183854566786,0.));
#9459=DIRECTION('',(0.,0.,-1.));
#9460=DIRECTION('',(0.,0.,-1.));
#9461=DIRECTION('',(-0.374606593415917,0.927183854566785,0.));
#9462=DIRECTION('',(-0.374606593415917,0.927183854566785,0.));
#9463=DIRECTION('',(0.,0.,1.));
#9464=DIRECTION('',(0.,0.,1.));
#9465=DIRECTION('',(0.,0.,-1.));
#9466=DIRECTION('center_axis',(-0.374606593415913,0.927183854566787,0.));
#9467=DIRECTION('ref_axis',(-0.927183854566787,-0.374606593415913,0.));
#9468=DIRECTION('center_axis',(0.374606593415913,-0.927183854566787,0.));
#9469=DIRECTION('ref_axis',(0.927183854566787,0.374606593415913,0.));
#9470=DIRECTION('center_axis',(-0.374606593415913,0.927183854566787,0.));
#9471=DIRECTION('ref_axis',(-0.927183854566787,-0.374606593415913,0.));
#9472=DIRECTION('center_axis',(-0.374606593415917,0.927183854566785,0.));
#9473=DIRECTION('ref_axis',(-0.927183854566785,-0.374606593415917,0.));
#9474=DIRECTION('',(0.927183854566785,0.374606593415917,0.));
#9475=DIRECTION('center_axis',(0.,0.,1.));
#9476=DIRECTION('ref_axis',(1.,0.,0.));
#9477=DIRECTION('center_axis',(0.374606593415917,-0.927183854566785,0.));
#9478=DIRECTION('ref_axis',(0.927183854566785,0.374606593415917,0.));
#9479=DIRECTION('',(0.927183854566785,0.374606593415917,0.));
#9480=DIRECTION('center_axis',(0.,0.,-1.));
#9481=DIRECTION('ref_axis',(1.,0.,0.));
#9482=DIRECTION('center_axis',(0.,0.,-1.));
#9483=DIRECTION('ref_axis',(-1.,0.,0.));
#11405=CARTESIAN_POINT('',(0.,0.,0.));
#11406=CARTESIAN_POINT('Origin',(22.,0.,3.));
#11407=CARTESIAN_POINT('',(23.5,-1.83697019872103E-16,4.));
#11408=CARTESIAN_POINT('Origin',(22.,0.,4.));
#11409=CARTESIAN_POINT('',(23.5,-1.83697019872103E-16,-1.));
#11410=CARTESIAN_POINT('',(23.5,-1.83697019872103E-16,3.));
#11411=CARTESIAN_POINT('Origin',(22.,0.,-1.));
#11412=CARTESIAN_POINT('Origin',(0.,0.,3.));
#11413=CARTESIAN_POINT('',(3.88651482573507,3.14563229086642,4.));
#11414=CARTESIAN_POINT('',(0.,-5.,4.));
#11415=CARTESIAN_POINT('Origin',(0.,0.,4.));
#11416=CARTESIAN_POINT('',(3.88651482573507,3.14563229086642,3.));
#11417=CARTESIAN_POINT('',(3.88651482573507,3.14563229086642,4.));
#11418=CARTESIAN_POINT('',(0.,5.,3.));
#11419=CARTESIAN_POINT('Origin',(0.,0.,3.));
#11420=CARTESIAN_POINT('',(0.,5.,0.));
#11421=CARTESIAN_POINT('',(0.,5.,3.));
#11422=CARTESIAN_POINT('',(3.88651482573507,3.14563229086642,0.));
#11423=CARTESIAN_POINT('Origin',(0.,0.,0.));
#11424=CARTESIAN_POINT('',(3.88651482573507,3.14563229086642,-1.));
#11425=CARTESIAN_POINT('',(3.88651482573507,3.14563229086642,-1.));
#11426=CARTESIAN_POINT('',(0.,-5.,-1.));
#11427=CARTESIAN_POINT('Origin',(0.,0.,-1.));
#11428=CARTESIAN_POINT('',(0.,-5.,3.));
#11429=CARTESIAN_POINT('Origin',(0.,0.,3.));
#11430=CARTESIAN_POINT('',(1.5,-1.83697019872103E-16,4.));
#11431=CARTESIAN_POINT('Origin',(0.,0.,4.));
#11432=CARTESIAN_POINT('',(1.5,-1.83697019872103E-16,-1.));
#11433=CARTESIAN_POINT('',(1.5,-1.83697019872103E-16,3.));
#11434=CARTESIAN_POINT('Origin',(0.,0.,-1.));
#11435=CARTESIAN_POINT('Origin',(0.,0.,4.));
#11436=CARTESIAN_POINT('',(45.2263053278443,6.62991522408338,4.));
#11437=CARTESIAN_POINT('',(45.4365685536382,6.10949547816422,4.));
#11438=CARTESIAN_POINT('',(45.2263053278443,6.62991522408338,4.));
#11439=CARTESIAN_POINT('',(54.708407099306,9.8555614123234,4.));
#11440=CARTESIAN_POINT('',(4.25411211450139,-10.5292969675612,4.));
#11441=CARTESIAN_POINT('',(52.2734642421026,15.8822564670075,4.));
#11442=CARTESIAN_POINT('',(55.4576202861379,8.00119370318982,4.));
#11443=CARTESIAN_POINT('',(20.7492131868318,3.14563229086643,4.));
#11444=CARTESIAN_POINT('',(20.7492131868318,3.14563229086643,4.));
#11445=CARTESIAN_POINT('',(22.7492131868318,3.14563229086642,4.));
#11446=CARTESIAN_POINT('',(22.,-5.,4.));
#11447=CARTESIAN_POINT('',(0.,-5.,4.));
#11448=CARTESIAN_POINT('',(26.8954874748715,-1.01695741473107,4.));
#11449=CARTESIAN_POINT('Origin',(22.,0.,4.));
#11450=CARTESIAN_POINT('',(29.9179419826634,2.60200444337179,4.));
#11451=CARTESIAN_POINT('Origin',(31.7909749497429,-2.03391482946214,4.));
#11452=CARTESIAN_POINT('',(42.622724431879,7.73506974638514,4.));
#11453=CARTESIAN_POINT('',(26.8147918762154,1.34825041766364,4.));
#11454=CARTESIAN_POINT('',(42.622724431879,7.73506974638514,4.));
#11455=CARTESIAN_POINT('Origin',(0.,0.,3.));
#11456=CARTESIAN_POINT('',(20.7492131868318,3.14563229086643,3.));
#11457=CARTESIAN_POINT('',(22.7492131868318,3.14563229086642,3.));
#11458=CARTESIAN_POINT('',(52.2734642421026,15.8822564670075,3.));
#11459=CARTESIAN_POINT('',(1.81916925729784,-4.50260191287694,3.));
#11460=CARTESIAN_POINT('',(51.5242510552708,17.7366241761411,3.));
#11461=CARTESIAN_POINT('',(50.4542949848047,20.3848583798845,3.));
#11462=CARTESIAN_POINT('',(20.,5.,3.));
#11463=CARTESIAN_POINT('',(1.06995607046601,-2.64823420374337,3.));
#11464=CARTESIAN_POINT('',(0.,5.,3.));
#11465=CARTESIAN_POINT('Origin',(0.,0.,-1.));
#11466=CARTESIAN_POINT('',(45.4365685536382,6.10949547816423,-1.));
#11467=CARTESIAN_POINT('',(54.708407099306,9.8555614123234,-1.));
#11468=CARTESIAN_POINT('',(4.25411211450139,-10.5292969675612,-1.));
#11469=CARTESIAN_POINT('',(45.2263053278443,6.62991522408338,-1.));
#11470=CARTESIAN_POINT('',(45.2263053278443,6.62991522408338,-1.));
#11471=CARTESIAN_POINT('',(42.622724431879,7.73506974638514,-1.));
#11472=CARTESIAN_POINT('',(42.622724431879,7.73506974638514,-1.));
#11473=CARTESIAN_POINT('',(29.9179419826634,2.60200444337179,-1.));
#11474=CARTESIAN_POINT('',(26.8147918762154,1.34825041766364,-1.));
#11475=CARTESIAN_POINT('',(26.8954874748715,-1.01695741473107,-1.));
#11476=CARTESIAN_POINT('Origin',(31.7909749497429,-2.03391482946214,-1.));
#11477=CARTESIAN_POINT('',(22.,-5.,-1.));
#11478=CARTESIAN_POINT('Origin',(22.,0.,-1.));
#11479=CARTESIAN_POINT('',(0.,-5.,-1.));
#11480=CARTESIAN_POINT('',(20.7492131868318,3.14563229086643,-1.));
#11481=CARTESIAN_POINT('',(22.7492131868318,3.14563229086642,-1.));
#11482=CARTESIAN_POINT('',(52.2734642421026,15.8822564670075,-1.));
#11483=CARTESIAN_POINT('',(20.7492131868318,3.14563229086643,-1.));
#11484=CARTESIAN_POINT('',(55.4576202861379,8.00119370318982,-1.));
#11485=CARTESIAN_POINT('Origin',(0.,0.,0.));
#11486=CARTESIAN_POINT('',(52.2734642421026,15.8822564670075,0.));
#11487=CARTESIAN_POINT('',(20.7492131868318,3.14563229086643,0.));
#11488=CARTESIAN_POINT('',(1.81916925729784,-4.50260191287694,0.));
#11489=CARTESIAN_POINT('',(22.7492131868318,3.14563229086642,0.));
#11490=CARTESIAN_POINT('',(20.,5.,0.));
#11491=CARTESIAN_POINT('',(0.,5.,0.));
#11492=CARTESIAN_POINT('',(51.5242510552708,17.7366241761411,0.));
#11493=CARTESIAN_POINT('',(1.06995607046601,-2.64823420374337,0.));
#11494=CARTESIAN_POINT('',(50.4542949848047,20.3848583798845,0.));
#11495=CARTESIAN_POINT('Origin',(22.7492131868318,3.14563229086642,4.));
#11496=CARTESIAN_POINT('',(20.7492131868318,3.14563229086643,4.));
#11497=CARTESIAN_POINT('Origin',(22.7492131868318,3.14563229086642,-1.));
#11498=CARTESIAN_POINT('',(20.7492131868318,3.14563229086643,-1.));
#11499=CARTESIAN_POINT('Origin',(0.,-5.,3.));
#11500=CARTESIAN_POINT('',(22.,-5.,3.));
#11501=CARTESIAN_POINT('Origin',(0.,5.,3.));
#11502=CARTESIAN_POINT('',(20.,5.,4.));
#11503=CARTESIAN_POINT('Origin',(22.,0.,3.));
#11504=CARTESIAN_POINT('',(26.8954874748715,-1.01695741473107,3.));
#11505=CARTESIAN_POINT('Origin',(3.29463570187568,-8.15450951250839,3.));
#11506=CARTESIAN_POINT('',(29.9179419826634,2.60200444337179,3.));
#11507=CARTESIAN_POINT('',(42.622724431879,7.73506974638514,3.));
#11508=CARTESIAN_POINT('Origin',(9.28931783023872,21.8842613872565,3.));
#11509=CARTESIAN_POINT('',(45.2263053278443,6.62991522408338,3.));
#11510=CARTESIAN_POINT('Origin',(41.1824564391369,16.6387924457253,3.));
#11511=CARTESIAN_POINT('',(45.4365685536382,6.10949547816422,-3.));
#11512=CARTESIAN_POINT('',(45.4365685536382,6.10949547816422,-3.));
#11513=CARTESIAN_POINT('',(46.18578174047,4.25512776903065,-3.));
#11514=CARTESIAN_POINT('',(41.1824564391368,16.6387924457254,-3.));
#11515=CARTESIAN_POINT('',(46.18578174047,4.25512776903065,6.));
#11516=CARTESIAN_POINT('',(46.18578174047,4.25512776903065,3.));
#11517=CARTESIAN_POINT('',(45.4365685536382,6.10949547816422,6.));
#11518=CARTESIAN_POINT('',(41.1824564391368,16.6387924457254,6.));
#11519=CARTESIAN_POINT('',(45.4365685536382,6.10949547816422,6.));
#11520=CARTESIAN_POINT('Origin',(5.00332530133316,-12.3836646766947,3.));
#11521=CARTESIAN_POINT('',(55.4576202861379,8.00119370318982,-3.));
#11522=CARTESIAN_POINT('',(5.00332530133317,-12.3836646766947,-3.));
#11523=CARTESIAN_POINT('',(55.4576202861379,8.00119370318982,6.));
#11524=CARTESIAN_POINT('',(55.4576202861379,8.00119370318982,3.));
#11525=CARTESIAN_POINT('',(5.00332530133317,-12.3836646766947,6.));
#11526=CARTESIAN_POINT('Origin',(50.4542949848047,20.3848583798845,3.));
#11527=CARTESIAN_POINT('',(52.2734642421026,15.8822564670075,4.));
#11528=CARTESIAN_POINT('',(54.708407099306,9.8555614123234,6.));
#11529=CARTESIAN_POINT('',(54.708407099306,9.8555614123234,6.));
#11530=CARTESIAN_POINT('',(50.4542949848046,20.3848583798846,6.));
#11531=CARTESIAN_POINT('',(54.708407099306,9.8555614123234,-3.));
#11532=CARTESIAN_POINT('',(50.4542949848046,20.3848583798846,-3.));
#11533=CARTESIAN_POINT('',(54.708407099306,9.8555614123234,-3.));
#11534=CARTESIAN_POINT('',(52.2734642421026,15.8822564670075,-1.));
#11535=CARTESIAN_POINT('',(51.5242510552708,17.7366241761411,3.));
#11536=CARTESIAN_POINT('Origin',(1.06995607046601,-2.64823420374337,3.));
#11537=CARTESIAN_POINT('Origin',(20.7492131868318,3.14563229086643,4.));
#11538=CARTESIAN_POINT('Origin',(20.7492131868318,3.14563229086643,-1.));
#11539=CARTESIAN_POINT('Origin',(4.25411211450139,-10.5292969675612,6.));
#11540=CARTESIAN_POINT('',(4.25411211450139,-10.5292969675612,6.));
#11541=CARTESIAN_POINT('Origin',(0.,0.,6.));
#11542=CARTESIAN_POINT('Origin',(4.25411211450139,-10.5292969675612,-3.));
#11543=CARTESIAN_POINT('',(4.25411211450139,-10.5292969675612,-3.));
#11544=CARTESIAN_POINT('Origin',(0.,0.,-3.));
#11545=CARTESIAN_POINT('Origin',(31.7909749497429,-2.03391482946214,3.));
#11917=UNCERTAINTY_MEASURE_WITH_UNIT(LENGTH_MEASURE(0.01),#11934,
'DISTANCE_ACCURACY_VALUE',
'Maximum model space distance between geometric entities at asserted c
onnectivities');
#11922=UNCERTAINTY_MEASURE_WITH_UNIT(LENGTH_MEASURE(0.01),#11934,
'DISTANCE_ACCURACY_VALUE',
'Maximum model space distance between geometric entities at asserted c
onnectivities');
#11928=(
GEOMETRIC_REPRESENTATION_CONTEXT(3)
GLOBAL_UNCERTAINTY_ASSIGNED_CONTEXT((#11917))
GLOBAL_UNIT_ASSIGNED_CONTEXT((#11934,#11936,#11937))
REPRESENTATION_CONTEXT('','3D')
);
#11933=(
GEOMETRIC_REPRESENTATION_CONTEXT(3)
GLOBAL_UNCERTAINTY_ASSIGNED_CONTEXT((#11922))
GLOBAL_UNIT_ASSIGNED_CONTEXT((#11934,#11936,#11937))
REPRESENTATION_CONTEXT('','3D')
);
#11934=(
LENGTH_UNIT()
NAMED_UNIT(*)
SI_UNIT(.MILLI.,.METRE.)
);
#11936=(
NAMED_UNIT(*)
PLANE_ANGLE_UNIT()
SI_UNIT($,.RADIAN.)
);
#11937=(
NAMED_UNIT(*)
SI_UNIT($,.STERADIAN.)
SOLID_ANGLE_UNIT()
);
#11943=SHAPE_DEFINITION_REPRESENTATION(#11953,#11992);
#11953=PRODUCT_DEFINITION_SHAPE('',$,#12003);
#11992=SHAPE_REPRESENTATION('',(#7448),#11928);
#11997=PRODUCT_DEFINITION_CONTEXT('part definition',#12029,'design');
#12003=PRODUCT_DEFINITION('Gripper Jaw','Gripper Jaw',#12013,#11997);
#12013=PRODUCT_DEFINITION_FORMATION('',$,#12036);
#12029=APPLICATION_CONTEXT(
'Core Data for Automotive Mechanical Design Process');
#12030=PRODUCT_CONTEXT('part definition',#12029,'mechanical');
#12036=PRODUCT('Gripper Jaw','Gripper Jaw',$,(#12030));
#12043=PRESENTATION_STYLE_ASSIGNMENT((#12047));
#12047=SURFACE_STYLE_USAGE(.BOTH.,#12051);
#12051=SURFACE_SIDE_STYLE('',(#12055));
#12055=SURFACE_STYLE_FILL_AREA(#12059);
#12059=FILL_AREA_STYLE('Opaque(61,176,222)',(#12063));
#12063=FILL_AREA_STYLE_COLOUR('Opaque(61,176,222)',#12067);
#12067=COLOUR_RGB('Opaque(61,176,222)',0.23921568627451,0.690196078431373,
0.870588235294118);
ENDSEC;
END-ISO-10303-21;
